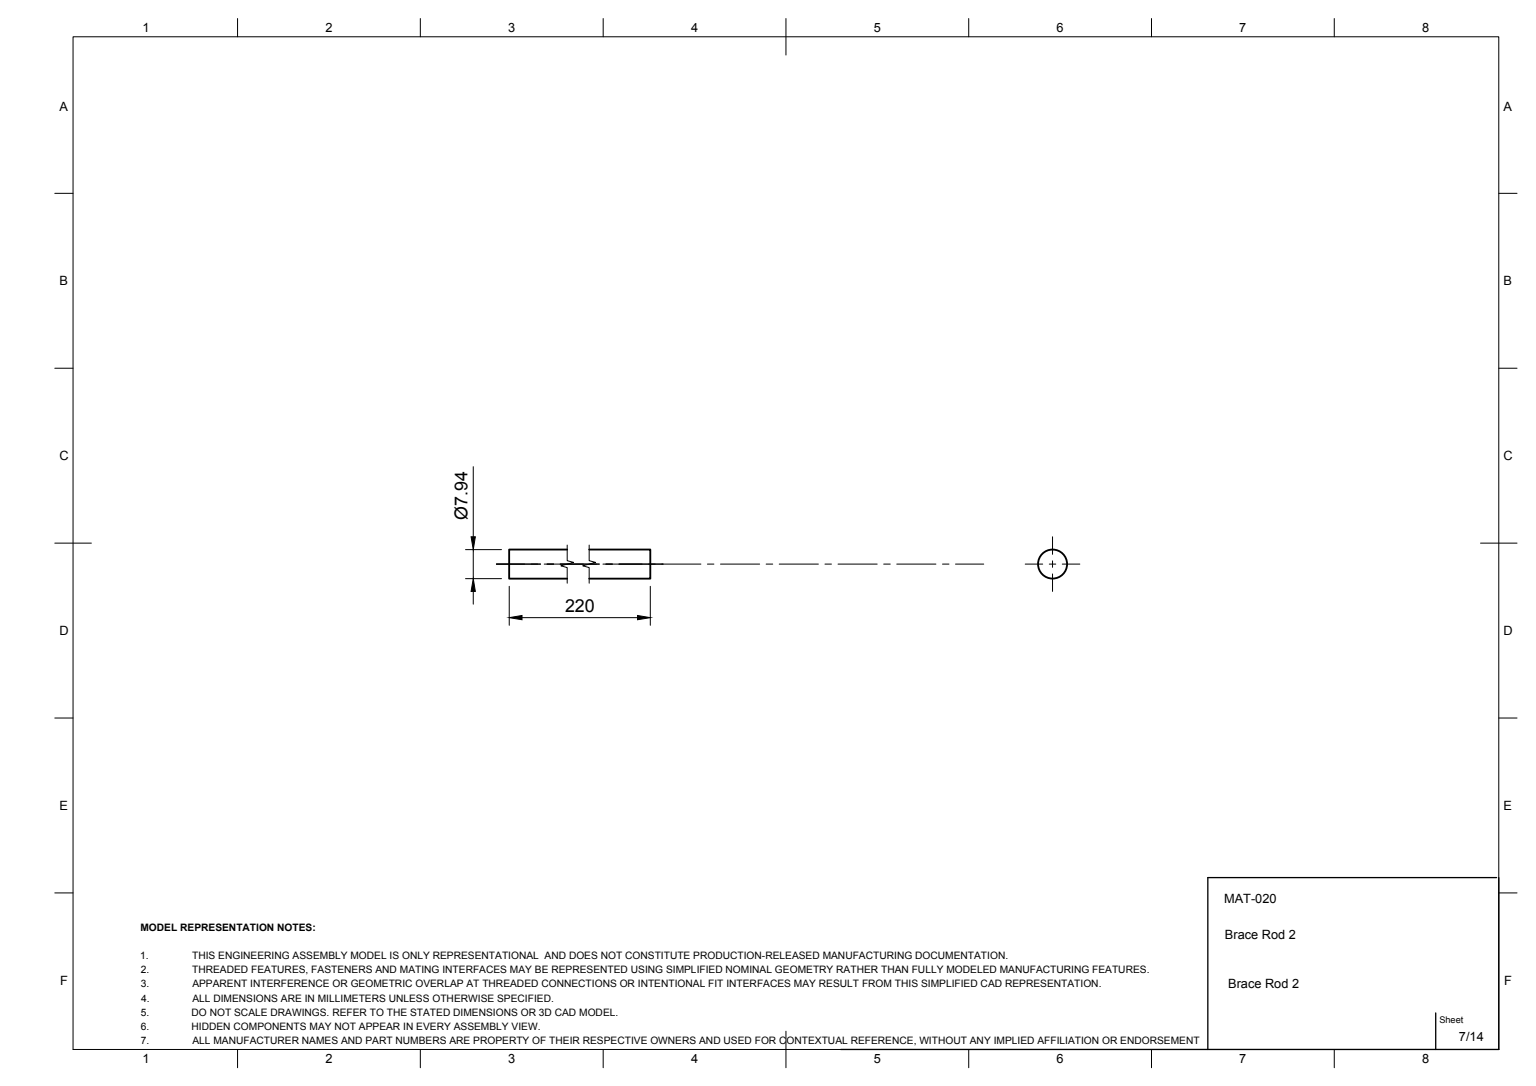
ISO-10303-21;
HEADER;
/* Generated by software containing ST-Developer
 * from STEP Tools, Inc. (www.steptools.com) 
 */

FILE_DESCRIPTION(
/* description */ ('STEP AP214'),
/* implementation_level */ '2;1');

FILE_NAME(
/* name */ 'Brace Rod 2.step',
/* time_stamp */ '2026-11-14T06:20:50-08:00',
/* author */ (''),
/* organization */ (''),
/* preprocessor_version */ 'ST-DEVELOPER v20.2',
/* originating_system */ 'Autodesk Translation Framework v15.17.0.0',
/* authorisation */ '');

FILE_SCHEMA (('AUTOMOTIVE_DESIGN { 1 0 10303 214 3 1 1 }'));
ENDSEC;

DATA;
#10=MECHANICAL_DESIGN_GEOMETRIC_PRESENTATION_REPRESENTATION('',(#958),#20658);
#395=PLANE('',#3811);
#396=PLANE('',#3812);
#449=LINE('',#5008,#642);
#642=VECTOR('',#4158,3.96875);
#835=CYLINDRICAL_SURFACE('',#3808,3.96875);
#934=SHAPE_REPRESENTATION_RELATIONSHIP('SRR','None',#20718,#946);
#946=ADVANCED_BREP_SHAPE_REPRESENTATION('',(#970),#20648);
#958=STYLED_ITEM('',(#20785),#970);
#970=MANIFOLD_SOLID_BREP('Body1',#3653);
#984=FACE_OUTER_BOUND('',#1193,.T.);
#985=FACE_OUTER_BOUND('',#1194,.T.);
#986=FACE_OUTER_BOUND('',#1195,.T.);
#1193=EDGE_LOOP('',(#2412,#2413,#2414,#2415));
#1194=EDGE_LOOP('',(#2416));
#1195=EDGE_LOOP('',(#2417));
#1425=CIRCLE('',#3809,3.96875);
#1426=CIRCLE('',#3810,3.96875);
#1549=VERTEX_POINT('',#5005);
#1550=VERTEX_POINT('',#5007);
#1888=EDGE_CURVE('',#1549,#1549,#1425,.T.);
#1889=EDGE_CURVE('',#1549,#1550,#449,.T.);
#1890=EDGE_CURVE('',#1550,#1550,#1426,.T.);
#2412=ORIENTED_EDGE('',*,*,#1888,.T.);
#2413=ORIENTED_EDGE('',*,*,#1889,.T.);
#2414=ORIENTED_EDGE('',*,*,#1890,.F.);
#2415=ORIENTED_EDGE('',*,*,#1889,.F.);
#2416=ORIENTED_EDGE('',*,*,#1890,.T.);
#2417=ORIENTED_EDGE('',*,*,#1888,.F.);
#3446=ADVANCED_FACE('',(#984),#835,.T.);
#3447=ADVANCED_FACE('',(#985),#395,.T.);
#3448=ADVANCED_FACE('',(#986),#396,.F.);
#3653=CLOSED_SHELL('',(#3446,#3447,#3448));
#3807=AXIS2_PLACEMENT_3D('',#5003,#4152,#4153);
#3808=AXIS2_PLACEMENT_3D('',#5004,#4154,#4155);
#3809=AXIS2_PLACEMENT_3D('',#5006,#4156,#4157);
#3810=AXIS2_PLACEMENT_3D('',#5009,#4159,#4160);
#3811=AXIS2_PLACEMENT_3D('',#5010,#4161,#4162);
#3812=AXIS2_PLACEMENT_3D('',#5011,#4163,#4164);
#4152=DIRECTION('axis',(0.,0.,1.));
#4153=DIRECTION('refdir',(1.,0.,0.));
#4154=DIRECTION('center_axis',(0.,0.,-1.));
#4155=DIRECTION('ref_axis',(-1.,0.,0.));
#4156=DIRECTION('center_axis',(0.,0.,1.));
#4157=DIRECTION('ref_axis',(1.,0.,0.));
#4158=DIRECTION('',(0.,0.,1.));
#4159=DIRECTION('center_axis',(0.,0.,1.));
#4160=DIRECTION('ref_axis',(1.,0.,0.));
#4161=DIRECTION('center_axis',(0.,0.,1.));
#4162=DIRECTION('ref_axis',(1.,0.,0.));
#4163=DIRECTION('center_axis',(0.,0.,1.));
#4164=DIRECTION('ref_axis',(1.,0.,0.));
#5003=CARTESIAN_POINT('',(0.,0.,0.));
#5004=CARTESIAN_POINT('Origin',(0.,0.,220.));
#5005=CARTESIAN_POINT('',(3.96875,-4.86031698411606E-16,0.));
#5006=CARTESIAN_POINT('Origin',(0.,0.,0.));
#5007=CARTESIAN_POINT('',(3.96875,-4.86031698411606E-16,220.));
#5008=CARTESIAN_POINT('',(3.96875,-4.86031698411606E-16,220.));
#5009=CARTESIAN_POINT('Origin',(0.,0.,220.));
#5010=CARTESIAN_POINT('Origin',(0.,0.,220.));
#5011=CARTESIAN_POINT('Origin',(0.,0.,0.));
#20634=UNCERTAINTY_MEASURE_WITH_UNIT(LENGTH_MEASURE(0.01),#20659,
'DISTANCE_ACCURACY_VALUE',
'Maximum model space distance between geometric entities at asserted c
onnectivities');
#20644=UNCERTAINTY_MEASURE_WITH_UNIT(LENGTH_MEASURE(0.01),#20659,
'DISTANCE_ACCURACY_VALUE',
'Maximum model space distance between geometric entities at asserted c
onnectivities');
#20648=(
GEOMETRIC_REPRESENTATION_CONTEXT(3)
GLOBAL_UNCERTAINTY_ASSIGNED_CONTEXT((#20634))
GLOBAL_UNIT_ASSIGNED_CONTEXT((#20659,#20661,#20662))
REPRESENTATION_CONTEXT('','3D')
);
#20658=(
GEOMETRIC_REPRESENTATION_CONTEXT(3)
GLOBAL_UNCERTAINTY_ASSIGNED_CONTEXT((#20644))
GLOBAL_UNIT_ASSIGNED_CONTEXT((#20659,#20661,#20662))
REPRESENTATION_CONTEXT('','3D')
);
#20659=(
LENGTH_UNIT()
NAMED_UNIT(*)
SI_UNIT(.MILLI.,.METRE.)
);
#20661=(
NAMED_UNIT(*)
PLANE_ANGLE_UNIT()
SI_UNIT($,.RADIAN.)
);
#20662=(
NAMED_UNIT(*)
SI_UNIT($,.STERADIAN.)
SOLID_ANGLE_UNIT()
);
#20666=SHAPE_DEFINITION_REPRESENTATION(#20679,#20718);
#20679=PRODUCT_DEFINITION_SHAPE('',$,#20732);
#20718=SHAPE_REPRESENTATION('',(#3807),#20648);
#20728=PRODUCT_DEFINITION_CONTEXT('part definition',#20769,'design');
#20732=PRODUCT_DEFINITION('Brace Rod 2','Brace Rod 2',#20745,#20728);
#20745=PRODUCT_DEFINITION_FORMATION('',$,#20774);
#20769=APPLICATION_CONTEXT(
'Core Data for Automotive Mechanical Design Process');
#20770=PRODUCT_CONTEXT('part definition',#20769,'mechanical');
#20774=PRODUCT('Brace Rod 2','Brace Rod 2',$,(#20770));
#20785=PRESENTATION_STYLE_ASSIGNMENT((#20790));
#20790=SURFACE_STYLE_USAGE(.BOTH.,#20795);
#20795=SURFACE_SIDE_STYLE('',(#20800));
#20800=SURFACE_STYLE_FILL_AREA(#20805);
#20805=FILL_AREA_STYLE('Opaque(97,158,199)',(#20810));
#20810=FILL_AREA_STYLE_COLOUR('Opaque(97,158,199)',#20815);
#20815=COLOUR_RGB('Opaque(97,158,199)',0.380392156862745,0.619607843137255,
0.780392156862745);
ENDSEC;
END-ISO-10303-21;
